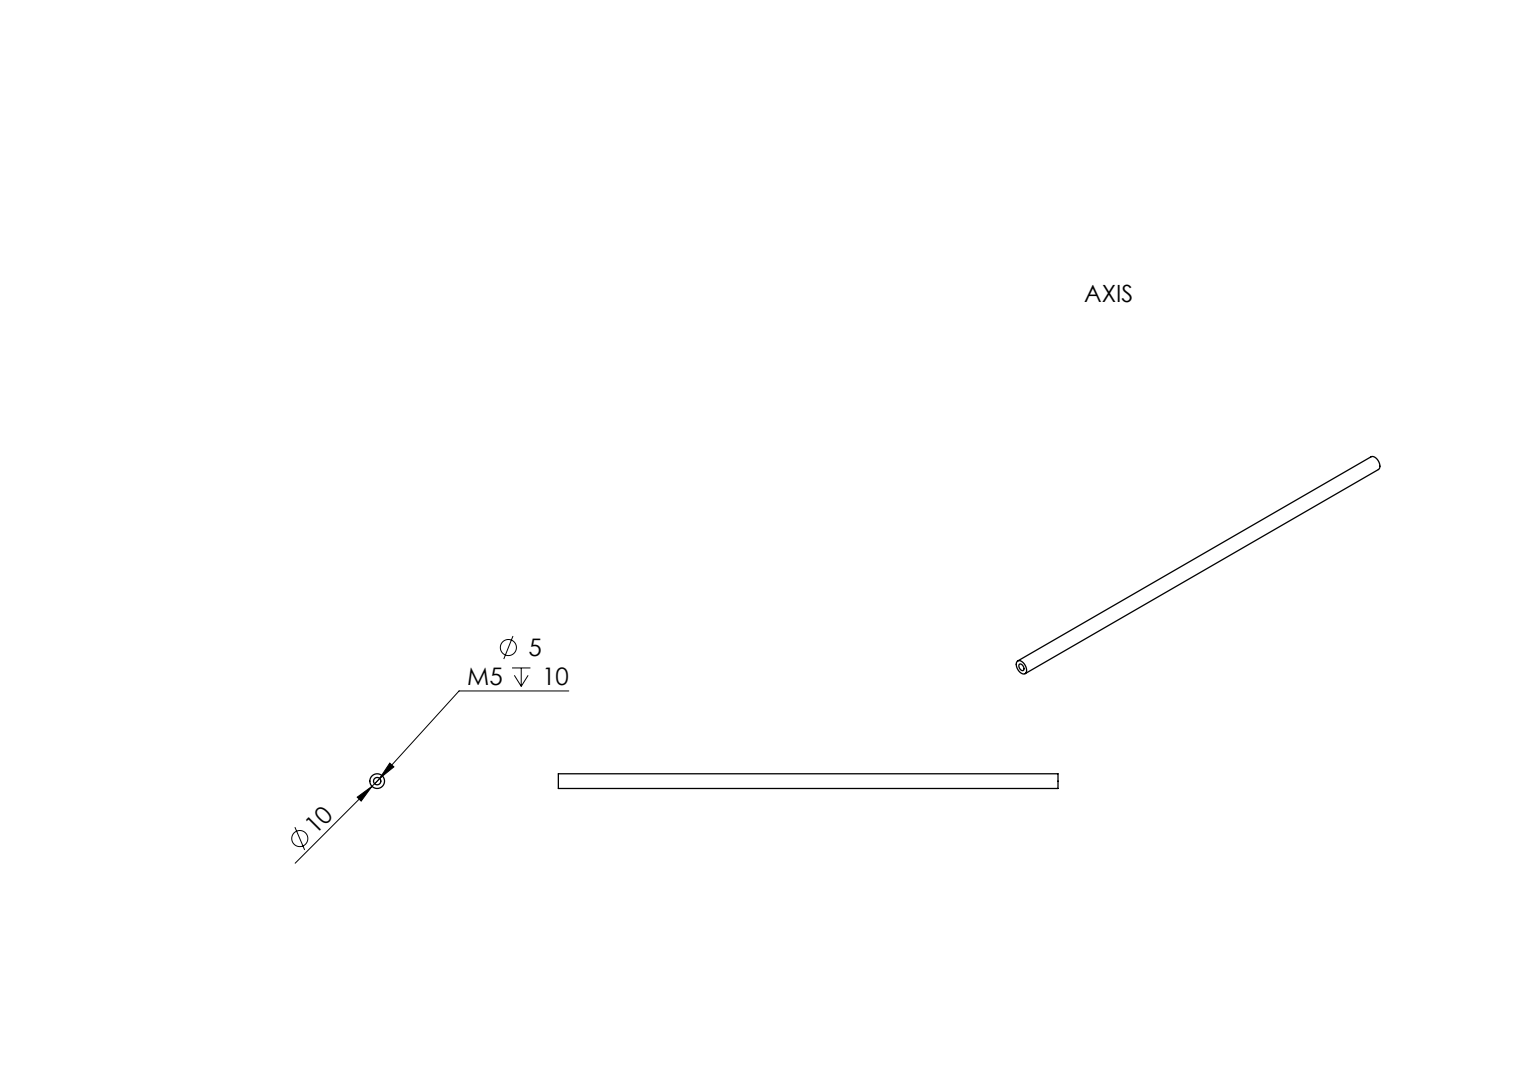
ISO-10303-21;
HEADER;
FILE_DESCRIPTION (('STEP AP214'),
    '1' );
FILE_NAME ('axis.step',
    '2026-10-24T13:33:06',
    ( '' ),
    ( '' ),
    'SwSTEP 2.0',
    'SolidWorks 2026',
    '' );
FILE_SCHEMA (( 'AUTOMOTIVE_DESIGN' ));
ENDSEC;

DATA;
#54=CARTESIAN_POINT ( 'NONE',  ( -299.9999999999999432, -75.00000000000008527, 329.9999999999999432 ) ) ;
#58=CARTESIAN_POINT ( 'NONE',  ( -297.4999999999999432, -75.00000000000008527, 10.00000000000000178 ) ) ;
#88=LINE ( 'NONE', #2296, #2370 ) ;
#150=LINE ( 'NONE', #1253, #5148 ) ;
#161=VERTEX_POINT ( 'NONE', #11045 ) ;
#187=( LENGTH_UNIT ( ) NAMED_UNIT ( * ) SI_UNIT ( .MILLI., .METRE. ) );
#200=CARTESIAN_POINT ( 'NONE',  ( -294.9999999999999432, -75.00000000000008527, 339.9999999999999432 ) ) ;
#241=AXIS2_PLACEMENT_3D ( 'NONE', #10628, #13202, #658 ) ;
#374=AXIS2_PLACEMENT_3D ( 'NONE', #11907, #9513, #3997 ) ;
#463=DIRECTION ( 'NONE',  ( -1.000000000000000000, 0.000000000000000000, 0.000000000000000000 ) ) ;
#493=SHAPE_DEFINITION_REPRESENTATION ( #2167, #7730 ) ;
#513=EDGE_LOOP ( 'NONE', ( #5449, #4903, #1270 ) ) ;
#542=CARTESIAN_POINT ( 'NONE',  ( -299.9999999999999432, -75.00000000000008527, 354.1421356237308942 ) ) ;
#553=EDGE_LOOP ( 'NONE', ( #2491, #10447 ) ) ;
#658=DIRECTION ( 'NONE',  ( -1.000000000000000000, 0.000000000000000000, 0.000000000000000000 ) ) ;
#671=ORIENTED_EDGE ( 'NONE', *, *, #14160, .F. ) ;
#702=MECHANICAL_DESIGN_GEOMETRIC_PRESENTATION_REPRESENTATION('',(#10000),#9500);
#727=DIRECTION ( 'NONE',  ( 1.000000000000000000, 0.000000000000000000, 0.000000000000000000 ) ) ;
#739=DIRECTION ( 'NONE',  ( -0.000000000000000000, -0.000000000000000000, 1.000000000000000000 ) ) ;
#837=ORIENTED_EDGE ( 'NONE', *, *, #9419, .F. ) ;
#869=LINE ( 'NONE', #935, #1336 ) ;
#891=ORIENTED_EDGE ( 'NONE', *, *, #9341, .F. ) ;
#902=CARTESIAN_POINT ( 'NONE',  ( 30.00000000000002842, -225.0000000000000000, 339.9999999999999432 ) ) ;
#929=DIRECTION ( 'NONE',  ( -0.000000000000000000, -0.000000000000000000, 1.000000000000000000 ) ) ;
#933=ORIENTED_EDGE ( 'NONE', *, *, #11083, .T. ) ;
#935=CARTESIAN_POINT ( 'NONE',  ( -294.9999999999999432, -75.00000000000008527, 354.1421356237308942 ) ) ;
#986=CARTESIAN_POINT ( 'NONE',  ( -299.9999999999999432, -75.00000000000008527, 11.50215154306610188 ) ) ;
#990=UNCERTAINTY_MEASURE_WITH_UNIT (LENGTH_MEASURE( 1.000000000000000082E-05 ), #187, 'distance_accuracy_value', 'NONE');
#997=FILL_AREA_STYLE_COLOUR ( '', #8873 ) ;
#1010=EDGE_LOOP ( 'NONE', ( #11631, #9599, #14024, #3706 ) ) ;
#1043=CIRCLE ( 'NONE', #374, 5.000000000000004441 ) ;
#1057=VECTOR ( 'NONE', #6494, 1000.000000000000000 ) ;
#1133=CIRCLE ( 'NONE', #9492, 2.500000000000002220 ) ;
#1135=DIRECTION ( 'NONE',  ( 1.000000000000000000, 0.000000000000000000, 0.000000000000000000 ) ) ;
#1142=SURFACE_STYLE_FILL_AREA ( #2394 ) ;
#1218=SHAPE_REPRESENTATION_RELATIONSHIP ( 'NONE' , 'NONE' ,  #7730, #6958 ) ;
#1253=CARTESIAN_POINT ( 'NONE',  ( -297.4999999999999432, -75.00000000000008527, 339.9999999999999432 ) ) ;
#1270=ORIENTED_EDGE ( 'NONE', *, *, #7944, .T. ) ;
#1294=CARTESIAN_POINT ( 'NONE',  ( -299.9999999999999432, -75.00000000000008527, 0.000000000000000000 ) ) ;
#1317=DIRECTION ( 'NONE',  ( -0.000000000000000000, -0.000000000000000000, -1.000000000000000000 ) ) ;
#1336=VECTOR ( 'NONE', #10698, 1000.000000000000000 ) ;
#1360=CYLINDRICAL_SURFACE ( 'NONE', #13582, 2.500000000000002220 ) ;
#1424=CONICAL_SURFACE ( 'NONE', #9083, 2.500000000000002220, 1.029744260000002631 ) ;
#1495=FACE_OUTER_BOUND ( 'NONE', #8735, .T. ) ;
#1502=ADVANCED_FACE ( 'NONE', ( #3222 ), #1424, .F. ) ;
#1583=AXIS2_PLACEMENT_3D ( 'NONE', #902, #8465, #6297 ) ;
#1611=FACE_OUTER_BOUND ( 'NONE', #2638, .T. ) ;
#1626=CARTESIAN_POINT ( 'NONE',  ( -302.4999999999999432, -75.00000000000008527, 329.9999999999999432 ) ) ;
#1664=ADVANCED_FACE ( 'NONE', ( #5875 ), #13416, .F. ) ;
#1685=LINE ( 'NONE', #12503, #3446 ) ;
#1806=CARTESIAN_POINT ( 'NONE',  ( -297.4999999999999432, -75.00000000000008527, 0.000000000000000000 ) ) ;
#1809=DIRECTION ( 'NONE',  ( -1.000000000000000000, 0.000000000000000000, 0.000000000000000000 ) ) ;
#1842=FACE_OUTER_BOUND ( 'NONE', #7097, .T. ) ;
#1850=VERTEX_POINT ( 'NONE', #7316 ) ;
#1900=VERTEX_POINT ( 'NONE', #986 ) ;
#1902=ORIENTED_EDGE ( 'NONE', *, *, #14091, .T. ) ;
#2074=CARTESIAN_POINT ( 'NONE',  ( -299.9999999999999432, -75.00000000000008527, 339.9999999999999432 ) ) ;
#2167=PRODUCT_DEFINITION_SHAPE ( 'NONE', 'NONE',  #5165 ) ;
#2242=EDGE_CURVE ( 'NONE', #161, #6979, #13421, .T. ) ;
#2251=SURFACE_SIDE_STYLE ('',( #1142 ) ) ;
#2286=DIRECTION ( 'NONE',  ( -0.000000000000000000, -0.000000000000000000, 1.000000000000000000 ) ) ;
#2296=CARTESIAN_POINT ( 'NONE',  ( -297.4999999999999432, -75.00000000000008527, 329.9999999999999432 ) ) ;
#2320=LINE ( 'NONE', #12259, #3984 ) ;
#2370=VECTOR ( 'NONE', #12374, 1000.000000000000000 ) ;
#2394=FILL_AREA_STYLE ('',( #997 ) ) ;
#2422=CARTESIAN_POINT ( 'NONE',  ( -302.4999999999999432, -75.00000000000008527, 0.000000000000000000 ) ) ;
#2491=ORIENTED_EDGE ( 'NONE', *, *, #9692, .F. ) ;
#2495=ORIENTED_EDGE ( 'NONE', *, *, #9341, .T. ) ;
#2597=AXIS2_PLACEMENT_3D ( 'NONE', #4504, #11241, #10287 ) ;
#2604=CARTESIAN_POINT ( 'NONE',  ( -299.9999999999999432, -75.00000000000008527, 10.00000000000000178 ) ) ;
#2638=EDGE_LOOP ( 'NONE', ( #671, #5749, #13109, #891 ) ) ;
#2669=FACE_OUTER_BOUND ( 'NONE', #513, .T. ) ;
#2702=AXIS2_PLACEMENT_3D ( 'NONE', #7505, #7288, #12947 ) ;
#2715=DIRECTION ( 'NONE',  ( -0.000000000000000000, -0.000000000000000000, 1.000000000000000000 ) ) ;
#2808=CARTESIAN_POINT ( 'NONE',  ( -299.9999999999999432, -75.00000000000008527, 339.9999999999999432 ) ) ;
#2858=DIRECTION ( 'NONE',  ( 1.000000000000000000, 0.000000000000000000, 0.000000000000000000 ) ) ;
#2903=ORIENTED_EDGE ( 'NONE', *, *, #9861, .F. ) ;
#2908=CARTESIAN_POINT ( 'NONE',  ( -299.9999999999999432, -75.00000000000008527, 0.000000000000000000 ) ) ;
#2919=VERTEX_POINT ( 'NONE', #4503 ) ;
#2968=CIRCLE ( 'NONE', #5503, 2.500000000000002220 ) ;
#3053=ORIENTED_EDGE ( 'NONE', *, *, #5851, .T. ) ;
#3091=CARTESIAN_POINT ( 'NONE',  ( -297.4999999999999432, -75.00000000000008527, 329.9999999999999432 ) ) ;
#3141=CARTESIAN_POINT ( 'NONE',  ( -299.9999999999999432, -75.00000000000008527, 0.000000000000000000 ) ) ;
#3222=FACE_OUTER_BOUND ( 'NONE', #8412, .T. ) ;
#3292=EDGE_LOOP ( 'NONE', ( #6661, #14147 ) ) ;
#3372=ADVANCED_FACE ( 'NONE', ( #13373 ), #13445, .T. ) ;
#3432=DIRECTION ( 'NONE',  ( -1.000000000000000000, 0.000000000000000000, 0.000000000000000000 ) ) ;
#3446=VECTOR ( 'NONE', #2715, 1000.000000000000000 ) ;
#3450=ORIENTED_EDGE ( 'NONE', *, *, #13548, .T. ) ;
#3459=PRODUCT ( 'axis', 'axis', '', ( #5025 ) ) ;
#3487=FACE_OUTER_BOUND ( 'NONE', #8187, .T. ) ;
#3504=DIRECTION ( 'NONE',  ( 0.000000000000000000, 0.000000000000000000, 1.000000000000000000 ) ) ;
#3523=DIRECTION ( 'NONE',  ( -1.000000000000000000, 0.000000000000000000, 0.000000000000000000 ) ) ;
#3550=ORIENTED_EDGE ( 'NONE', *, *, #13548, .F. ) ;
#3606=ORIENTED_EDGE ( 'NONE', *, *, #10135, .T. ) ;
#3662=DIRECTION ( 'NONE',  ( 1.000000000000000000, 0.000000000000000000, 0.000000000000000000 ) ) ;
#3667=VERTEX_POINT ( 'NONE', #3091 ) ;
#3693=FACE_OUTER_BOUND ( 'NONE', #6504, .T. ) ;
#3694=DIRECTION ( 'NONE',  ( 1.000000000000000000, 0.000000000000000000, 0.000000000000000000 ) ) ;
#3706=ORIENTED_EDGE ( 'NONE', *, *, #9692, .T. ) ;
#3823=MANIFOLD_SOLID_BREP ( 'AdvancedHole2', #5223 ) ;
#3875=DIRECTION ( 'NONE',  ( -0.000000000000000000, -0.000000000000000000, 1.000000000000000000 ) ) ;
#3984=VECTOR ( 'NONE', #5654, 1000.000000000000000 ) ;
#3997=DIRECTION ( 'NONE',  ( -1.000000000000000000, 0.000000000000000000, 0.000000000000000000 ) ) ;
#4131=FACE_OUTER_BOUND ( 'NONE', #10936, .T. ) ;
#4211=( GEOMETRIC_REPRESENTATION_CONTEXT ( 3 ) GLOBAL_UNCERTAINTY_ASSIGNED_CONTEXT ( ( #990 ) ) GLOBAL_UNIT_ASSIGNED_CONTEXT ( ( #187, #6680, #11243 ) ) REPRESENTATION_CONTEXT ( 'NONE', 'WORKASPACE' ) );
#4323=CIRCLE ( 'NONE', #8007, 2.500000000000002220 ) ;
#4355=AXIS2_PLACEMENT_3D ( 'NONE', #3141, #5522, #4369 ) ;
#4369=DIRECTION ( 'NONE',  ( 1.000000000000000000, 0.000000000000000000, 0.000000000000000000 ) ) ;
#4392=ADVANCED_FACE ( 'NONE', ( #5154, #4131 ), #6372, .F. ) ;
#4503=CARTESIAN_POINT ( 'NONE',  ( -299.9999999999999432, -75.00000000000008527, 328.4978484569338661 ) ) ;
#4504=CARTESIAN_POINT ( 'NONE',  ( -299.9999999999999432, -75.00000000000008527, 10.00000000000000178 ) ) ;
#4519=DIRECTION ( 'NONE',  ( 1.000000000000000000, 0.000000000000000000, -0.000000000000000000 ) ) ;
#4538=DIRECTION ( 'NONE',  ( -0.000000000000000000, -0.000000000000000000, -1.000000000000000000 ) ) ;
#4734=FACE_OUTER_BOUND ( 'NONE', #3292, .T. ) ;
#4898=EDGE_CURVE ( 'NONE', #1850, #7429, #1133, .T. ) ;
#4903=ORIENTED_EDGE ( 'NONE', *, *, #13930, .T. ) ;
#4907=EDGE_CURVE ( 'NONE', #161, #11376, #8957, .T. ) ;
#4938=( GEOMETRIC_REPRESENTATION_CONTEXT ( 3 ) GLOBAL_UNCERTAINTY_ASSIGNED_CONTEXT ( ( #6530 ) ) GLOBAL_UNIT_ASSIGNED_CONTEXT ( ( #7539, #5176, #10753 ) ) REPRESENTATION_CONTEXT ( 'NONE', 'WORKASPACE' ) );
#4949=CARTESIAN_POINT ( 'NONE',  ( -302.4999999999999432, -75.00000000000008527, 10.00000000000000178 ) ) ;
#4997=CARTESIAN_POINT ( 'NONE',  ( -294.9999999999999432, -75.00000000000008527, 0.000000000000000000 ) ) ;
#5009=CIRCLE ( 'NONE', #13102, 2.500000000000002220 ) ;
#5025=PRODUCT_CONTEXT ( 'NONE', #12581, 'mechanical' ) ;
#5044=DIRECTION ( 'NONE',  ( -1.000000000000000000, 0.000000000000000000, 0.000000000000000000 ) ) ;
#5077=DIRECTION ( 'NONE',  ( 1.000000000000000000, 0.000000000000000000, 0.000000000000000000 ) ) ;
#5096=FACE_OUTER_BOUND ( 'NONE', #5827, .T. ) ;
#5148=VECTOR ( 'NONE', #2286, 1000.000000000000000 ) ;
#5154=FACE_BOUND ( 'NONE', #13746, .T. ) ;
#5165=PRODUCT_DEFINITION ( 'UNKNOWN', '', #5409, #9636 ) ;
#5176=( NAMED_UNIT ( * ) PLANE_ANGLE_UNIT ( ) SI_UNIT ( $, .RADIAN. ) );
#5223=CLOSED_SHELL ( 'NONE', ( #9787, #12921, #10489, #9524, #10020, #6916, #3372, #4392, #6411, #1502, #1664, #8664 ) ) ;
#5327=DIRECTION ( 'NONE',  ( -0.000000000000000000, -0.000000000000000000, 1.000000000000000000 ) ) ;
#5409=PRODUCT_DEFINITION_FORMATION_WITH_SPECIFIED_SOURCE ( 'ANY', '', #3459, .NOT_KNOWN. ) ;
#5449=ORIENTED_EDGE ( 'NONE', *, *, #11834, .F. ) ;
#5503=AXIS2_PLACEMENT_3D ( 'NONE', #11169, #11105, #1135 ) ;
#5522=DIRECTION ( 'NONE',  ( 0.000000000000000000, 0.000000000000000000, 1.000000000000000000 ) ) ;
#5654=DIRECTION ( 'NONE',  ( -0.000000000000000000, -0.000000000000000000, -1.000000000000000000 ) ) ;
#5749=ORIENTED_EDGE ( 'NONE', *, *, #13390, .T. ) ;
#5827=EDGE_LOOP ( 'NONE', ( #9158, #9805, #933, #2903 ) ) ;
#5837=AXIS2_PLACEMENT_3D ( 'NONE', #13583, #3875, #3662 ) ;
#5851=EDGE_CURVE ( 'NONE', #11376, #8753, #6204, .T. ) ;
#5875=FACE_OUTER_BOUND ( 'NONE', #1010, .T. ) ;
#6204=CIRCLE ( 'NONE', #4355, 5.000000000000004441 ) ;
#6218=VECTOR ( 'NONE', #10930, 1000.000000000000000 ) ;
#6297=DIRECTION ( 'NONE',  ( -1.000000000000000000, 0.000000000000000000, 0.000000000000000000 ) ) ;
#6372=PLANE ( 'NONE',  #1583 ) ;
#6411=ADVANCED_FACE ( 'NONE', ( #1495 ), #1360, .F. ) ;
#6494=DIRECTION ( 'NONE',  ( 0.8571673013836870192, 1.049727191973306873E-16, -0.5150380737757234151 ) ) ;
#6502=CARTESIAN_POINT ( 'NONE',  ( -304.9999999999999432, -75.00000000000008527, 354.1421356237308942 ) ) ;
#6504=EDGE_LOOP ( 'NONE', ( #7133, #3450, #11412, #13954 ) ) ;
#6530=UNCERTAINTY_MEASURE_WITH_UNIT (LENGTH_MEASURE( 1.000000000000000082E-05 ), #7539, 'distance_accuracy_value', 'NONE');
#6551=VERTEX_POINT ( 'NONE', #2422 ) ;
#6641=CONICAL_SURFACE ( 'NONE', #11772, 2.500000000000002220, 1.029744260000002631 ) ;
#6661=ORIENTED_EDGE ( 'NONE', *, *, #5851, .F. ) ;
#6680=( NAMED_UNIT ( * ) PLANE_ANGLE_UNIT ( ) SI_UNIT ( $, .RADIAN. ) );
#6735=EDGE_CURVE ( 'NONE', #3667, #9074, #5009, .T. ) ;
#6740=CARTESIAN_POINT ( 'NONE',  ( -302.4999999999999432, -75.00000000000008527, 339.9999999999999432 ) ) ;
#6763=AXIS2_PLACEMENT_3D ( 'NONE', #14062, #8553, #10883 ) ;
#6837=ORIENTED_EDGE ( 'NONE', *, *, #11911, .F. ) ;
#6843=EDGE_CURVE ( 'NONE', #8753, #11376, #7305, .T. ) ;
#6916=ADVANCED_FACE ( 'NONE', ( #9006, #4734 ), #7971, .F. ) ;
#6925=VERTEX_POINT ( 'NONE', #58 ) ;
#6958=ADVANCED_BREP_SHAPE_REPRESENTATION ( '', ( #3823, #14039 ), #4938 ) ;
#6976=( NAMED_UNIT ( * ) SI_UNIT ( $, .STERADIAN. ) SOLID_ANGLE_UNIT ( ) );
#6979=VERTEX_POINT ( 'NONE', #200 ) ;
#7047=( LENGTH_UNIT ( ) NAMED_UNIT ( * ) SI_UNIT ( .MILLI., .METRE. ) );
#7097=EDGE_LOOP ( 'NONE', ( #8330, #8023, #13248 ) ) ;
#7098=VERTEX_POINT ( 'NONE', #8338 ) ;
#7133=ORIENTED_EDGE ( 'NONE', *, *, #2242, .T. ) ;
#7288=DIRECTION ( 'NONE',  ( -0.000000000000000000, -0.000000000000000000, 1.000000000000000000 ) ) ;
#7296=APPLICATION_CONTEXT ( 'automotive_design' ) ;
#7305=CIRCLE ( 'NONE', #13095, 5.000000000000004441 ) ;
#7316=CARTESIAN_POINT ( 'NONE',  ( -297.4999999999999432, -75.00000000000008527, 339.9999999999999432 ) ) ;
#7345=VECTOR ( 'NONE', #13707, 1000.000000000000000 ) ;
#7429=VERTEX_POINT ( 'NONE', #6740 ) ;
#7502=CARTESIAN_POINT ( 'NONE',  ( -299.9999999999999432, -75.00000000000008527, 329.9999999999999432 ) ) ;
#7505=CARTESIAN_POINT ( 'NONE',  ( -299.9999999999999432, -75.00000000000008527, 339.9999999999999432 ) ) ;
#7539=( LENGTH_UNIT ( ) NAMED_UNIT ( * ) SI_UNIT ( .MILLI., .METRE. ) );
#7579=ORIENTED_EDGE ( 'NONE', *, *, #4898, .T. ) ;
#7722=CARTESIAN_POINT ( 'NONE',  ( -299.9999999999999432, -75.00000000000008527, 354.1421356237308942 ) ) ;
#7730=SHAPE_REPRESENTATION ( 'axis', ( #14039 ), #4938 ) ;
#7944=EDGE_CURVE ( 'NONE', #7098, #6925, #4323, .T. ) ;
#7971=PLANE ( 'NONE',  #10097 ) ;
#8007=AXIS2_PLACEMENT_3D ( 'NONE', #9462, #11706, #5044 ) ;
#8023=ORIENTED_EDGE ( 'NONE', *, *, #9419, .T. ) ;
#8086=AXIS2_PLACEMENT_3D ( 'NONE', #2074, #12089, #9915 ) ;
#8125=VECTOR ( 'NONE', #11490, 1000.000000000000000 ) ;
#8142=LINE ( 'NONE', #12582, #8125 ) ;
#8187=EDGE_LOOP ( 'NONE', ( #12635, #12104, #14047 ) ) ;
#8197=( NAMED_UNIT ( * ) PLANE_ANGLE_UNIT ( ) SI_UNIT ( $, .RADIAN. ) );
#8282=ORIENTED_EDGE ( 'NONE', *, *, #6735, .T. ) ;
#8330=ORIENTED_EDGE ( 'NONE', *, *, #10135, .F. ) ;
#8338=CARTESIAN_POINT ( 'NONE',  ( -302.4999999999999432, -75.00000000000008527, 10.00000000000000178 ) ) ;
#8412=EDGE_LOOP ( 'NONE', ( #837, #3606, #8282 ) ) ;
#8465=DIRECTION ( 'NONE',  ( 0.000000000000000000, 0.000000000000000000, -1.000000000000000000 ) ) ;
#8494=ORIENTED_EDGE ( 'NONE', *, *, #4898, .F. ) ;
#8552=ORIENTED_EDGE ( 'NONE', *, *, #2242, .F. ) ;
#8553=DIRECTION ( 'NONE',  ( -0.000000000000000000, -0.000000000000000000, -1.000000000000000000 ) ) ;
#8643=MECHANICAL_DESIGN_GEOMETRIC_PRESENTATION_REPRESENTATION('',(#13038),#4211);
#8664=ADVANCED_FACE ( 'NONE', ( #2669 ), #6641, .F. ) ;
#8735=EDGE_LOOP ( 'NONE', ( #13219, #10907, #2495, #7579 ) ) ;
#8748=AXIS2_PLACEMENT_3D ( 'NONE', #2908, #11757, #1809 ) ;
#8753=VERTEX_POINT ( 'NONE', #4997 ) ;
#8873=COLOUR_RGB ( '',0.8941176470588234615, 0.8941176470588234615, 0.8941176470588234615 ) ;
#8957=LINE ( 'NONE', #6502, #6218 ) ;
#9006=FACE_BOUND ( 'NONE', #553, .T. ) ;
#9074=VERTEX_POINT ( 'NONE', #1626 ) ;
#9083=AXIS2_PLACEMENT_3D ( 'NONE', #54, #929, #2858 ) ;
#9128=CARTESIAN_POINT ( 'NONE',  ( -299.9999999999999432, -75.00000000000008527, 10.00000000000000178 ) ) ;
#9158=ORIENTED_EDGE ( 'NONE', *, *, #14294, .F. ) ;
#9173=LINE ( 'NONE', #13021, #1057 ) ;
#9341=EDGE_CURVE ( 'NONE', #3667, #1850, #150, .T. ) ;
#9388=CYLINDRICAL_SURFACE ( 'NONE', #5837, 2.500000000000002220 ) ;
#9418=DIRECTION ( 'NONE',  ( 0.000000000000000000, 0.000000000000000000, 1.000000000000000000 ) ) ;
#9419=EDGE_CURVE ( 'NONE', #2919, #9074, #8142, .T. ) ;
#9462=CARTESIAN_POINT ( 'NONE',  ( -299.9999999999999432, -75.00000000000008527, 10.00000000000000178 ) ) ;
#9492=AXIS2_PLACEMENT_3D ( 'NONE', #2808, #10720, #13815 ) ;
#9500=( GEOMETRIC_REPRESENTATION_CONTEXT ( 3 ) GLOBAL_UNCERTAINTY_ASSIGNED_CONTEXT ( ( #9679 ) ) GLOBAL_UNIT_ASSIGNED_CONTEXT ( ( #7047, #8197, #6976 ) ) REPRESENTATION_CONTEXT ( 'NONE', 'WORKASPACE' ) );
#9513=DIRECTION ( 'NONE',  ( 0.000000000000000000, 0.000000000000000000, -1.000000000000000000 ) ) ;
#9524=ADVANCED_FACE ( 'NONE', ( #1611 ), #9388, .F. ) ;
#9599=ORIENTED_EDGE ( 'NONE', *, *, #7944, .F. ) ;
#9605=DIRECTION ( 'NONE',  ( 0.000000000000000000, 0.000000000000000000, 1.000000000000000000 ) ) ;
#9636=PRODUCT_DEFINITION_CONTEXT ( 'detailed design', #7296, 'design' ) ;
#9679=UNCERTAINTY_MEASURE_WITH_UNIT (LENGTH_MEASURE( 1.000000000000000082E-05 ), #7047, 'distance_accuracy_value', 'NONE');
#9692=EDGE_CURVE ( 'NONE', #6551, #11920, #11402, .T. ) ;
#9765=CARTESIAN_POINT ( 'NONE',  ( -297.4999999999999432, -75.00000000000008527, 0.000000000000000000 ) ) ;
#9787=ADVANCED_FACE ( 'NONE', ( #3487 ), #10466, .F. ) ;
#9805=ORIENTED_EDGE ( 'NONE', *, *, #10934, .T. ) ;
#9861=EDGE_CURVE ( 'NONE', #7098, #6551, #2320, .T. ) ;
#9914=AXIS2_PLACEMENT_3D ( 'NONE', #2604, #13472, #463 ) ;
#9915=DIRECTION ( 'NONE',  ( -1.000000000000000000, 0.000000000000000000, 0.000000000000000000 ) ) ;
#10000=STYLED_ITEM('',(#14396),#3823);
#10020=ADVANCED_FACE ( 'NONE', ( #3693 ), #12606, .T. ) ;
#10097=AXIS2_PLACEMENT_3D ( 'NONE', #13496, #3504, #4519 ) ;
#10135=EDGE_CURVE ( 'NONE', #2919, #3667, #88, .T. ) ;
#10287=DIRECTION ( 'NONE',  ( -1.000000000000000000, 0.000000000000000000, 0.000000000000000000 ) ) ;
#10365=CIRCLE ( 'NONE', #9914, 2.500000000000002220 ) ;
#10447=ORIENTED_EDGE ( 'NONE', *, *, #11083, .F. ) ;
#10466=CONICAL_SURFACE ( 'NONE', #2597, 2.500000000000002220, 1.029744260000002631 ) ;
#10489=ADVANCED_FACE ( 'NONE', ( #1842 ), #13271, .F. ) ;
#10508=CARTESIAN_POINT ( 'NONE',  ( 0.000000000000000000, 0.000000000000000000, 0.000000000000000000 ) ) ;
#10509=DIRECTION ( 'NONE',  ( -0.000000000000000000, -0.000000000000000000, -1.000000000000000000 ) ) ;
#10512=CARTESIAN_POINT ( 'NONE',  ( -299.9999999999999432, -75.00000000000008527, 339.9999999999999432 ) ) ;
#10628=CARTESIAN_POINT ( 'NONE',  ( -299.9999999999999432, -75.00000000000008527, 0.000000000000000000 ) ) ;
#10675=CYLINDRICAL_SURFACE ( 'NONE', #8748, 2.500000000000002220 ) ;
#10696=CARTESIAN_POINT ( 'NONE',  ( -299.9999999999999432, -75.00000000000008527, 0.000000000000000000 ) ) ;
#10698=DIRECTION ( 'NONE',  ( -0.000000000000000000, -0.000000000000000000, -1.000000000000000000 ) ) ;
#10720=DIRECTION ( 'NONE',  ( -0.000000000000000000, -0.000000000000000000, 1.000000000000000000 ) ) ;
#10753=( NAMED_UNIT ( * ) SI_UNIT ( $, .STERADIAN. ) SOLID_ANGLE_UNIT ( ) );
#10883=DIRECTION ( 'NONE',  ( -1.000000000000000000, 0.000000000000000000, 0.000000000000000000 ) ) ;
#10907=ORIENTED_EDGE ( 'NONE', *, *, #6735, .F. ) ;
#10930=DIRECTION ( 'NONE',  ( -0.000000000000000000, -0.000000000000000000, -1.000000000000000000 ) ) ;
#10934=EDGE_CURVE ( 'NONE', #6925, #11920, #12833, .T. ) ;
#10936=EDGE_LOOP ( 'NONE', ( #8552, #12464 ) ) ;
#11045=CARTESIAN_POINT ( 'NONE',  ( -304.9999999999999432, -75.00000000000008527, 339.9999999999999432 ) ) ;
#11083=EDGE_CURVE ( 'NONE', #11920, #6551, #13018, .T. ) ;
#11105=DIRECTION ( 'NONE',  ( -0.000000000000000000, -0.000000000000000000, 1.000000000000000000 ) ) ;
#11169=CARTESIAN_POINT ( 'NONE',  ( -299.9999999999999432, -75.00000000000008527, 329.9999999999999432 ) ) ;
#11241=DIRECTION ( 'NONE',  ( -0.000000000000000000, -0.000000000000000000, -1.000000000000000000 ) ) ;
#11243=( NAMED_UNIT ( * ) SI_UNIT ( $, .STERADIAN. ) SOLID_ANGLE_UNIT ( ) );
#11376=VERTEX_POINT ( 'NONE', #14255 ) ;
#11380=DIRECTION ( 'NONE',  ( -1.000000000000000000, 0.000000000000000000, 0.000000000000000000 ) ) ;
#11396=DIRECTION ( 'NONE',  ( -0.000000000000000000, -0.000000000000000000, -1.000000000000000000 ) ) ;
#11402=CIRCLE ( 'NONE', #241, 2.500000000000002220 ) ;
#11412=ORIENTED_EDGE ( 'NONE', *, *, #6843, .T. ) ;
#11424=AXIS2_PLACEMENT_3D ( 'NONE', #7502, #739, #12727 ) ;
#11459=EDGE_LOOP ( 'NONE', ( #3550, #1902, #13094, #3053 ) ) ;
#11490=DIRECTION ( 'NONE',  ( -0.8571673013836870192, 1.049727191973306873E-16, 0.5150380737757234151 ) ) ;
#11524=DIRECTION ( 'NONE',  ( -0.000000000000000000, -0.000000000000000000, -1.000000000000000000 ) ) ;
#11631=ORIENTED_EDGE ( 'NONE', *, *, #10934, .F. ) ;
#11706=DIRECTION ( 'NONE',  ( -0.000000000000000000, -0.000000000000000000, -1.000000000000000000 ) ) ;
#11757=DIRECTION ( 'NONE',  ( -0.000000000000000000, -0.000000000000000000, -1.000000000000000000 ) ) ;
#11772=AXIS2_PLACEMENT_3D ( 'NONE', #9128, #10509, #11380 ) ;
#11834=EDGE_CURVE ( 'NONE', #1900, #6925, #9173, .T. ) ;
#11835=AXIS2_PLACEMENT_3D ( 'NONE', #7722, #4538, #3523 ) ;
#11871=AXIS2_PLACEMENT_3D ( 'NONE', #542, #11524, #12751 ) ;
#11907=CARTESIAN_POINT ( 'NONE',  ( -299.9999999999999432, -75.00000000000008527, 339.9999999999999432 ) ) ;
#11911=EDGE_CURVE ( 'NONE', #7429, #1850, #14271, .T. ) ;
#11920=VERTEX_POINT ( 'NONE', #9765 ) ;
#12089=DIRECTION ( 'NONE',  ( 0.000000000000000000, 0.000000000000000000, -1.000000000000000000 ) ) ;
#12104=ORIENTED_EDGE ( 'NONE', *, *, #11834, .T. ) ;
#12109=AXIS2_PLACEMENT_3D ( 'NONE', #1294, #11396, #3432 ) ;
#12184=PRESENTATION_STYLE_ASSIGNMENT (( #13408 ) ) ;
#12259=CARTESIAN_POINT ( 'NONE',  ( -302.4999999999999432, -75.00000000000008527, 0.000000000000000000 ) ) ;
#12355=VECTOR ( 'NONE', #1317, 1000.000000000000000 ) ;
#12374=DIRECTION ( 'NONE',  ( 0.8571673013836870192, 0.000000000000000000, 0.5150380737757234151 ) ) ;
#12464=ORIENTED_EDGE ( 'NONE', *, *, #14091, .F. ) ;
#12503=CARTESIAN_POINT ( 'NONE',  ( -302.4999999999999432, -75.00000000000008527, 339.9999999999999432 ) ) ;
#12581=APPLICATION_CONTEXT ( 'automotive_design' ) ;
#12582=CARTESIAN_POINT ( 'NONE',  ( -302.4999999999999432, -75.00000000000008527, 329.9999999999999432 ) ) ;
#12606=CYLINDRICAL_SURFACE ( 'NONE', #11871, 5.000000000000004441 ) ;
#12635=ORIENTED_EDGE ( 'NONE', *, *, #13930, .F. ) ;
#12727=DIRECTION ( 'NONE',  ( 1.000000000000000000, 0.000000000000000000, 0.000000000000000000 ) ) ;
#12751=DIRECTION ( 'NONE',  ( -1.000000000000000000, 0.000000000000000000, 0.000000000000000000 ) ) ;
#12833=LINE ( 'NONE', #1806, #12355 ) ;
#12921=ADVANCED_FACE ( 'NONE', ( #5096 ), #10675, .F. ) ;
#12947=DIRECTION ( 'NONE',  ( 1.000000000000000000, 0.000000000000000000, 0.000000000000000000 ) ) ;
#13018=CIRCLE ( 'NONE', #6763, 2.500000000000002220 ) ;
#13021=CARTESIAN_POINT ( 'NONE',  ( -297.4999999999999432, -75.00000000000008527, 10.00000000000000178 ) ) ;
#13038=STYLED_ITEM ( 'NONE', ( #12184 ), #6958 ) ;
#13094=ORIENTED_EDGE ( 'NONE', *, *, #4907, .T. ) ;
#13095=AXIS2_PLACEMENT_3D ( 'NONE', #10696, #9605, #14010 ) ;
#13102=AXIS2_PLACEMENT_3D ( 'NONE', #13146, #5327, #727 ) ;
#13109=ORIENTED_EDGE ( 'NONE', *, *, #11911, .T. ) ;
#13146=CARTESIAN_POINT ( 'NONE',  ( -299.9999999999999432, -75.00000000000008527, 329.9999999999999432 ) ) ;
#13202=DIRECTION ( 'NONE',  ( -0.000000000000000000, -0.000000000000000000, -1.000000000000000000 ) ) ;
#13219=ORIENTED_EDGE ( 'NONE', *, *, #13390, .F. ) ;
#13248=ORIENTED_EDGE ( 'NONE', *, *, #14160, .T. ) ;
#13271=CONICAL_SURFACE ( 'NONE', #11424, 2.500000000000002220, 1.029744260000002631 ) ;
#13373=FACE_OUTER_BOUND ( 'NONE', #11459, .T. ) ;
#13390=EDGE_CURVE ( 'NONE', #9074, #7429, #1685, .T. ) ;
#13408=SURFACE_STYLE_USAGE ( .BOTH. , #2251 ) ;
#13416=CYLINDRICAL_SURFACE ( 'NONE', #12109, 2.500000000000002220 ) ;
#13421=CIRCLE ( 'NONE', #8086, 5.000000000000004441 ) ;
#13445=CYLINDRICAL_SURFACE ( 'NONE', #11835, 5.000000000000004441 ) ;
#13472=DIRECTION ( 'NONE',  ( -0.000000000000000000, -0.000000000000000000, -1.000000000000000000 ) ) ;
#13496=CARTESIAN_POINT ( 'NONE',  ( -299.9999999999999432, -75.00000000000008527, 0.000000000000000000 ) ) ;
#13548=EDGE_CURVE ( 'NONE', #6979, #8753, #869, .T. ) ;
#13582=AXIS2_PLACEMENT_3D ( 'NONE', #10512, #13692, #3694 ) ;
#13583=CARTESIAN_POINT ( 'NONE',  ( -299.9999999999999432, -75.00000000000008527, 339.9999999999999432 ) ) ;
#13692=DIRECTION ( 'NONE',  ( -0.000000000000000000, -0.000000000000000000, 1.000000000000000000 ) ) ;
#13707=DIRECTION ( 'NONE',  ( -0.8571673013836870192, 0.000000000000000000, -0.5150380737757234151 ) ) ;
#13746=EDGE_LOOP ( 'NONE', ( #8494, #6837 ) ) ;
#13779=LINE ( 'NONE', #4949, #7345 ) ;
#13815=DIRECTION ( 'NONE',  ( 1.000000000000000000, 0.000000000000000000, 0.000000000000000000 ) ) ;
#13930=EDGE_CURVE ( 'NONE', #1900, #7098, #13779, .T. ) ;
#13954=ORIENTED_EDGE ( 'NONE', *, *, #4907, .F. ) ;
#14010=DIRECTION ( 'NONE',  ( 1.000000000000000000, 0.000000000000000000, 0.000000000000000000 ) ) ;
#14024=ORIENTED_EDGE ( 'NONE', *, *, #9861, .T. ) ;
#14039=AXIS2_PLACEMENT_3D ( 'NONE', #10508, #9418, #5077 ) ;
#14047=ORIENTED_EDGE ( 'NONE', *, *, #14294, .T. ) ;
#14062=CARTESIAN_POINT ( 'NONE',  ( -299.9999999999999432, -75.00000000000008527, 0.000000000000000000 ) ) ;
#14091=EDGE_CURVE ( 'NONE', #6979, #161, #1043, .T. ) ;
#14147=ORIENTED_EDGE ( 'NONE', *, *, #6843, .F. ) ;
#14160=EDGE_CURVE ( 'NONE', #9074, #3667, #2968, .T. ) ;
#14255=CARTESIAN_POINT ( 'NONE',  ( -304.9999999999999432, -75.00000000000008527, 0.000000000000000000 ) ) ;
#14271=CIRCLE ( 'NONE', #2702, 2.500000000000002220 ) ;
#14294=EDGE_CURVE ( 'NONE', #6925, #7098, #10365, .T. ) ;
#14390=COLOUR_RGB('Light Blue',0.38,0.62,0.78);
#14391=FILL_AREA_STYLE_COLOUR('',#14390);
#14392=FILL_AREA_STYLE('',(#14391));
#14393=SURFACE_STYLE_FILL_AREA(#14392);
#14394=SURFACE_SIDE_STYLE('',(#14393));
#14395=SURFACE_STYLE_USAGE(.BOTH.,#14394);
#14396=PRESENTATION_STYLE_ASSIGNMENT((#14395));
ENDSEC;
END-ISO-10303-21;
